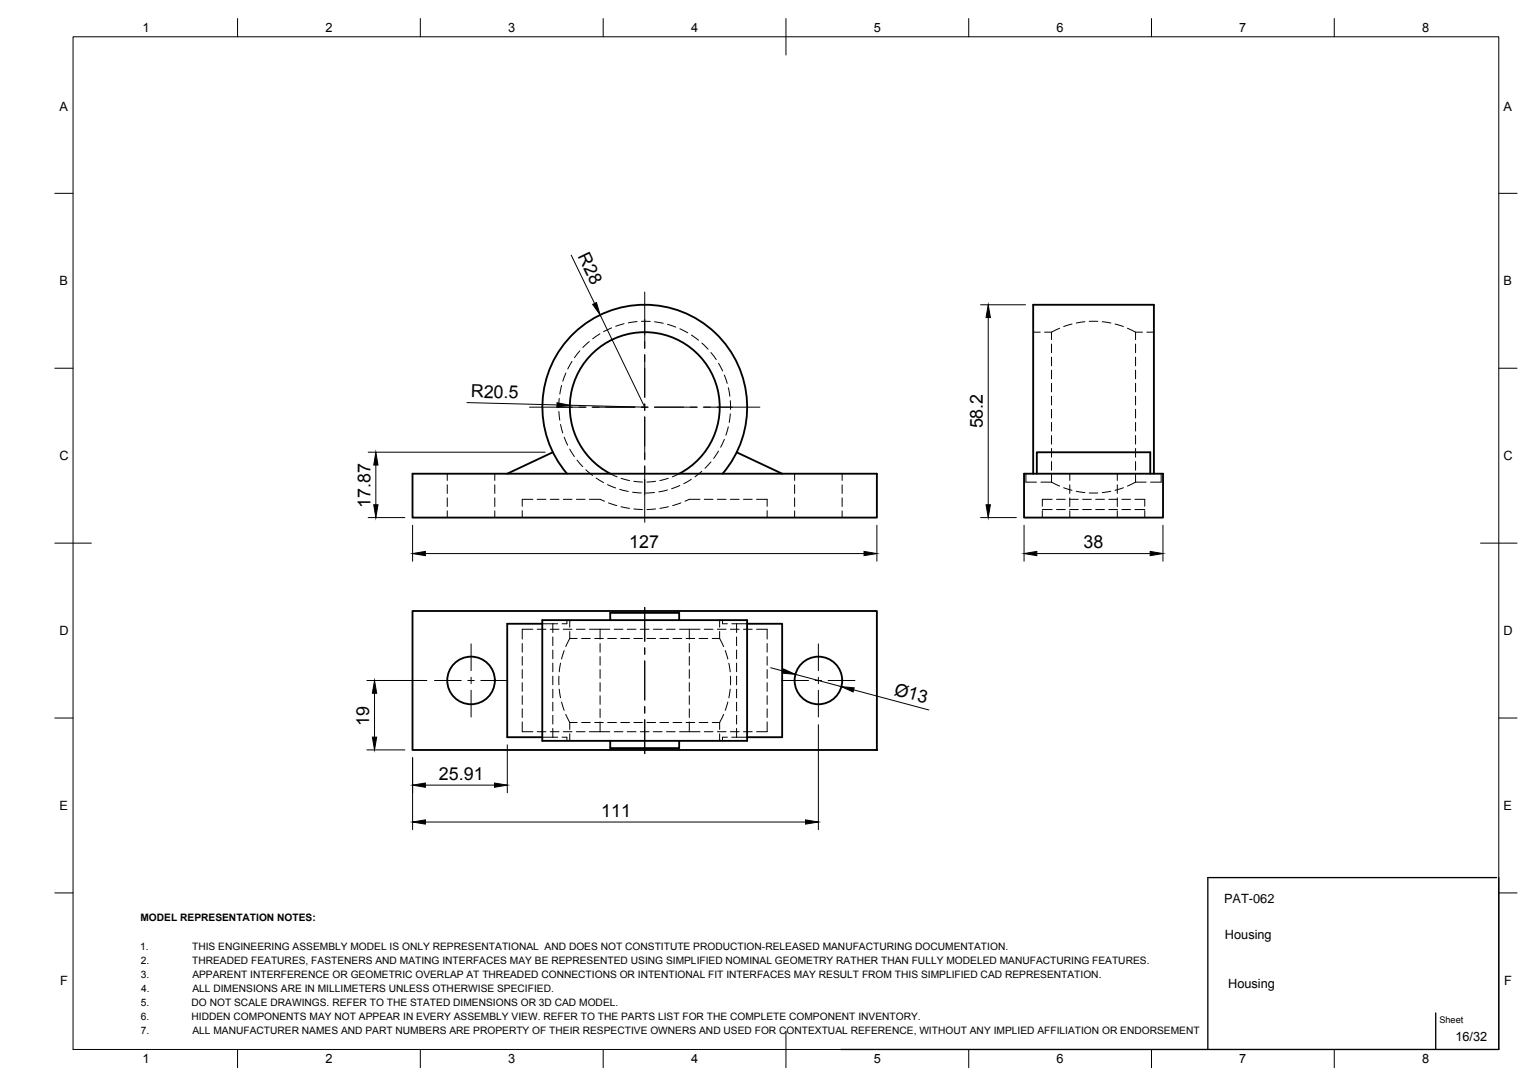
ISO-10303-21;
HEADER;
/* Generated by software containing ST-Developer
 * from STEP Tools, Inc. (www.steptools.com) 
 */

FILE_DESCRIPTION(
/* description */ ('Jaw-coupled motor to shaft test stand'),
/* implementation_level */ '2;1');

FILE_NAME(
/* name */ 'Housing.step',
/* time_stamp */ '2026-10-27T10:46:06-07:00',
/* author */ (''),
/* organization */ (''),
/* preprocessor_version */ 'ST-DEVELOPER v20.2',
/* originating_system */ 'Autodesk Translation Framework v15.17.0.0',
/* authorisation */ '');

FILE_SCHEMA (('AUTOMOTIVE_DESIGN { 1 0 10303 214 3 1 1 }'));
ENDSEC;

DATA;
#10=MECHANICAL_DESIGN_GEOMETRIC_PRESENTATION_REPRESENTATION('',(#353),#19361);
#274=SPHERICAL_SURFACE('',#11594,2.35);
#289=SHAPE_REPRESENTATION_RELATIONSHIP('SRR','None',#19504,#321);
#321=ADVANCED_BREP_SHAPE_REPRESENTATION('',(#386),#19340);
#353=STYLED_ITEM('',(#19725),#386);
#386=MANIFOLD_SOLID_BREP('Body1',#10997);
#452=FACE_BOUND('',#1817,.T.);
#453=FACE_BOUND('',#1818,.T.);
#454=FACE_BOUND('',#1826,.T.);
#455=FACE_BOUND('',#1827,.T.);
#456=FACE_BOUND('',#1828,.T.);
#457=FACE_BOUND('',#1845,.T.);
#458=FACE_BOUND('',#1846,.T.);
#459=FACE_BOUND('',#1847,.T.);
#601=PLANE('',#11580);
#602=PLANE('',#11591);
#603=PLANE('',#11592);
#604=PLANE('',#11596);
#605=PLANE('',#11598);
#606=PLANE('',#11600);
#607=PLANE('',#11602);
#608=PLANE('',#11603);
#609=PLANE('',#11605);
#610=PLANE('',#11606);
#611=PLANE('',#11614);
#612=PLANE('',#11615);
#613=PLANE('',#11616);
#614=PLANE('',#11617);
#615=PLANE('',#11618);
#616=PLANE('',#11619);
#617=PLANE('',#11620);
#618=PLANE('',#11625);
#619=PLANE('',#11626);
#620=PLANE('',#11627);
#621=PLANE('',#11628);
#622=PLANE('',#11629);
#1142=FACE_OUTER_BOUND('',#1811,.T.);
#1143=FACE_OUTER_BOUND('',#1812,.T.);
#1144=FACE_OUTER_BOUND('',#1813,.T.);
#1145=FACE_OUTER_BOUND('',#1814,.T.);
#1146=FACE_OUTER_BOUND('',#1815,.T.);
#1147=FACE_OUTER_BOUND('',#1816,.T.);
#1148=FACE_OUTER_BOUND('',#1819,.T.);
#1149=FACE_OUTER_BOUND('',#1820,.T.);
#1150=FACE_OUTER_BOUND('',#1821,.T.);
#1151=FACE_OUTER_BOUND('',#1822,.T.);
#1152=FACE_OUTER_BOUND('',#1823,.T.);
#1153=FACE_OUTER_BOUND('',#1824,.T.);
#1154=FACE_OUTER_BOUND('',#1825,.T.);
#1155=FACE_OUTER_BOUND('',#1829,.T.);
#1156=FACE_OUTER_BOUND('',#1830,.T.);
#1157=FACE_OUTER_BOUND('',#1831,.T.);
#1158=FACE_OUTER_BOUND('',#1832,.T.);
#1159=FACE_OUTER_BOUND('',#1833,.T.);
#1160=FACE_OUTER_BOUND('',#1834,.T.);
#1161=FACE_OUTER_BOUND('',#1835,.T.);
#1162=FACE_OUTER_BOUND('',#1836,.T.);
#1163=FACE_OUTER_BOUND('',#1837,.T.);
#1164=FACE_OUTER_BOUND('',#1838,.T.);
#1165=FACE_OUTER_BOUND('',#1839,.T.);
#1166=FACE_OUTER_BOUND('',#1840,.T.);
#1167=FACE_OUTER_BOUND('',#1841,.T.);
#1168=FACE_OUTER_BOUND('',#1842,.T.);
#1169=FACE_OUTER_BOUND('',#1843,.T.);
#1170=FACE_OUTER_BOUND('',#1844,.T.);
#1811=EDGE_LOOP('',(#7832,#7833));
#1812=EDGE_LOOP('',(#7834,#7835,#7836,#7837,#7838,#7839,#7840,#7841));
#1813=EDGE_LOOP('',(#7842,#7843,#7844,#7845,#7846,#7847,#7848,#7849));
#1814=EDGE_LOOP('',(#7850,#7851));
#1815=EDGE_LOOP('',(#7852,#7853,#7854,#7855,#7856));
#1816=EDGE_LOOP('',(#7857,#7858));
#1817=EDGE_LOOP('',(#7859));
#1818=EDGE_LOOP('',(#7860));
#1819=EDGE_LOOP('',(#7861,#7862,#7863));
#1820=EDGE_LOOP('',(#7864,#7865,#7866));
#1821=EDGE_LOOP('',(#7867,#7868,#7869));
#1822=EDGE_LOOP('',(#7870,#7871,#7872,#7873));
#1823=EDGE_LOOP('',(#7874,#7875,#7876));
#1824=EDGE_LOOP('',(#7877,#7878,#7879,#7880));
#1825=EDGE_LOOP('',(#7881,#7882,#7883,#7884));
#1826=EDGE_LOOP('',(#7885,#7886,#7887,#7888,#7889,#7890,#7891,#7892,#7893,
#7894,#7895,#7896,#7897,#7898,#7899,#7900,#7901,#7902,#7903,#7904));
#1827=EDGE_LOOP('',(#7905));
#1828=EDGE_LOOP('',(#7906));
#1829=EDGE_LOOP('',(#7907,#7908,#7909,#7910));
#1830=EDGE_LOOP('',(#7911,#7912,#7913,#7914,#7915,#7916,#7917,#7918,#7919,
#7920,#7921,#7922));
#1831=EDGE_LOOP('',(#7923,#7924,#7925,#7926,#7927));
#1832=EDGE_LOOP('',(#7928,#7929,#7930,#7931,#7932,#7933));
#1833=EDGE_LOOP('',(#7934,#7935,#7936,#7937));
#1834=EDGE_LOOP('',(#7938,#7939,#7940,#7941));
#1835=EDGE_LOOP('',(#7942,#7943,#7944,#7945,#7946,#7947));
#1836=EDGE_LOOP('',(#7948,#7949,#7950,#7951));
#1837=EDGE_LOOP('',(#7952,#7953,#7954,#7955));
#1838=EDGE_LOOP('',(#7956,#7957,#7958,#7959));
#1839=EDGE_LOOP('',(#7960,#7961,#7962,#7963));
#1840=EDGE_LOOP('',(#7964,#7965,#7966,#7967));
#1841=EDGE_LOOP('',(#7968,#7969,#7970,#7971));
#1842=EDGE_LOOP('',(#7972,#7973,#7974,#7975));
#1843=EDGE_LOOP('',(#7976,#7977,#7978,#7979));
#1844=EDGE_LOOP('',(#7980,#7981,#7982,#7983));
#1845=EDGE_LOOP('',(#7984,#7985,#7986,#7987));
#1846=EDGE_LOOP('',(#7988));
#1847=EDGE_LOOP('',(#7989));
#2548=LINE('',#15972,#3701);
#2549=LINE('',#15977,#3702);
#2550=LINE('',#15981,#3703);
#2551=LINE('',#15985,#3704);
#2552=LINE('',#15992,#3705);
#2553=LINE('',#15995,#3706);
#2554=LINE('',#15997,#3707);
#2555=LINE('',#16000,#3708);
#2556=LINE('',#16003,#3709);
#2557=LINE('',#16006,#3710);
#2558=LINE('',#16014,#3711);
#2559=LINE('',#16016,#3712);
#2560=LINE('',#16021,#3713);
#2561=LINE('',#16024,#3714);
#2562=LINE('',#16028,#3715);
#2563=LINE('',#16031,#3716);
#2564=LINE('',#16033,#3717);
#2565=LINE('',#16034,#3718);
#2566=LINE('',#16038,#3719);
#2567=LINE('',#16040,#3720);
#2568=LINE('',#16043,#3721);
#2569=LINE('',#16044,#3722);
#2570=LINE('',#16048,#3723);
#2571=LINE('',#16050,#3724);
#2572=LINE('',#16052,#3725);
#2573=LINE('',#16053,#3726);
#2574=LINE('',#16054,#3727);
#2575=LINE('',#16056,#3728);
#2576=LINE('',#16057,#3729);
#2577=LINE('',#16059,#3730);
#2578=LINE('',#16060,#3731);
#2579=LINE('',#16061,#3732);
#2580=LINE('',#16071,#3733);
#2581=LINE('',#16074,#3734);
#2582=LINE('',#16080,#3735);
#2583=LINE('',#16082,#3736);
#2584=LINE('',#16084,#3737);
#2585=LINE('',#16086,#3738);
#2586=LINE('',#16087,#3739);
#2587=LINE('',#16090,#3740);
#2588=LINE('',#16091,#3741);
#2589=LINE('',#16094,#3742);
#2590=LINE('',#16096,#3743);
#2591=LINE('',#16097,#3744);
#2592=LINE('',#16099,#3745);
#2593=LINE('',#16101,#3746);
#2594=LINE('',#16102,#3747);
#2595=LINE('',#16104,#3748);
#2596=LINE('',#16109,#3749);
#2597=LINE('',#16113,#3750);
#2598=LINE('',#16117,#3751);
#2599=LINE('',#16118,#3752);
#2600=LINE('',#16119,#3753);
#2601=LINE('',#16122,#3754);
#2602=LINE('',#16123,#3755);
#2603=LINE('',#16126,#3756);
#2604=LINE('',#16127,#3757);
#2605=LINE('',#16129,#3758);
#3701=VECTOR('',#12929,1.);
#3702=VECTOR('',#12934,1.);
#3703=VECTOR('',#12937,1.);
#3704=VECTOR('',#12940,2.05);
#3705=VECTOR('',#12949,2.05);
#3706=VECTOR('',#12952,1.);
#3707=VECTOR('',#12953,1.);
#3708=VECTOR('',#12958,1.);
#3709=VECTOR('',#12961,1.);
#3710=VECTOR('',#12964,1.);
#3711=VECTOR('',#12971,1.);
#3712=VECTOR('',#12972,1.);
#3713=VECTOR('',#12977,1.);
#3714=VECTOR('',#12980,1.);
#3715=VECTOR('',#12983,1.);
#3716=VECTOR('',#12986,1.);
#3717=VECTOR('',#12989,1.);
#3718=VECTOR('',#12990,1.);
#3719=VECTOR('',#12993,1.);
#3720=VECTOR('',#12994,1.);
#3721=VECTOR('',#12999,1.);
#3722=VECTOR('',#13000,1.);
#3723=VECTOR('',#13003,1.);
#3724=VECTOR('',#13004,1.);
#3725=VECTOR('',#13005,1.);
#3726=VECTOR('',#13006,1.);
#3727=VECTOR('',#13007,1.);
#3728=VECTOR('',#13008,1.);
#3729=VECTOR('',#13009,1.);
#3730=VECTOR('',#13010,1.);
#3731=VECTOR('',#13011,1.);
#3732=VECTOR('',#13012,1.);
#3733=VECTOR('',#13021,1.);
#3734=VECTOR('',#13024,1.);
#3735=VECTOR('',#13033,1.);
#3736=VECTOR('',#13034,1.);
#3737=VECTOR('',#13035,1.);
#3738=VECTOR('',#13036,1.);
#3739=VECTOR('',#13037,1.);
#3740=VECTOR('',#13040,1.);
#3741=VECTOR('',#13041,1.);
#3742=VECTOR('',#13044,1.);
#3743=VECTOR('',#13045,1.);
#3744=VECTOR('',#13046,1.);
#3745=VECTOR('',#13049,1.);
#3746=VECTOR('',#13050,1.);
#3747=VECTOR('',#13051,1.);
#3748=VECTOR('',#13054,1.);
#3749=VECTOR('',#13061,0.65);
#3750=VECTOR('',#13066,0.65);
#3751=VECTOR('',#13069,1.);
#3752=VECTOR('',#13070,1.);
#3753=VECTOR('',#13071,1.);
#3754=VECTOR('',#13074,1.);
#3755=VECTOR('',#13075,1.);
#3756=VECTOR('',#13078,1.);
#3757=VECTOR('',#13079,1.);
#3758=VECTOR('',#13082,1.);
#4751=CIRCLE('',#11581,2.05);
#4752=CIRCLE('',#11583,2.05);
#4753=CIRCLE('',#11584,2.05);
#4754=CIRCLE('',#11585,2.05);
#4755=CIRCLE('',#11586,2.05);
#4756=CIRCLE('',#11588,2.05);
#4757=CIRCLE('',#11589,2.05);
#4758=CIRCLE('',#11590,2.05);
#4759=CIRCLE('',#11593,2.8);
#4760=CIRCLE('',#11595,2.35);
#4761=CIRCLE('',#11597,2.8);
#4762=CIRCLE('',#11599,2.8);
#4763=CIRCLE('',#11601,2.8);
#4764=CIRCLE('',#11604,2.8);
#4765=CIRCLE('',#11607,0.65);
#4766=CIRCLE('',#11608,0.65);
#4767=CIRCLE('',#11610,2.8);
#4768=CIRCLE('',#11611,2.8);
#4769=CIRCLE('',#11613,2.8);
#4770=CIRCLE('',#11622,0.65);
#4771=CIRCLE('',#11624,0.65);
#5105=VERTEX_POINT('',#15970);
#5106=VERTEX_POINT('',#15971);
#5107=VERTEX_POINT('',#15975);
#5108=VERTEX_POINT('',#15976);
#5109=VERTEX_POINT('',#15978);
#5110=VERTEX_POINT('',#15980);
#5111=VERTEX_POINT('',#15982);
#5112=VERTEX_POINT('',#15984);
#5113=VERTEX_POINT('',#15989);
#5114=VERTEX_POINT('',#15991);
#5115=VERTEX_POINT('',#15993);
#5116=VERTEX_POINT('',#15996);
#5117=VERTEX_POINT('',#16002);
#5118=VERTEX_POINT('',#16004);
#5119=VERTEX_POINT('',#16008);
#5120=VERTEX_POINT('',#16009);
#5121=VERTEX_POINT('',#16012);
#5122=VERTEX_POINT('',#16013);
#5123=VERTEX_POINT('',#16015);
#5124=VERTEX_POINT('',#16019);
#5125=VERTEX_POINT('',#16020);
#5126=VERTEX_POINT('',#16022);
#5127=VERTEX_POINT('',#16026);
#5128=VERTEX_POINT('',#16027);
#5129=VERTEX_POINT('',#16029);
#5130=VERTEX_POINT('',#16036);
#5131=VERTEX_POINT('',#16037);
#5132=VERTEX_POINT('',#16039);
#5133=VERTEX_POINT('',#16046);
#5134=VERTEX_POINT('',#16047);
#5135=VERTEX_POINT('',#16049);
#5136=VERTEX_POINT('',#16051);
#5137=VERTEX_POINT('',#16055);
#5138=VERTEX_POINT('',#16058);
#5139=VERTEX_POINT('',#16062);
#5140=VERTEX_POINT('',#16064);
#5141=VERTEX_POINT('',#16067);
#5142=VERTEX_POINT('',#16068);
#5143=VERTEX_POINT('',#16070);
#5144=VERTEX_POINT('',#16072);
#5145=VERTEX_POINT('',#16079);
#5146=VERTEX_POINT('',#16081);
#5147=VERTEX_POINT('',#16083);
#5148=VERTEX_POINT('',#16085);
#5149=VERTEX_POINT('',#16089);
#5150=VERTEX_POINT('',#16093);
#5151=VERTEX_POINT('',#16095);
#5152=VERTEX_POINT('',#16100);
#5153=VERTEX_POINT('',#16107);
#5154=VERTEX_POINT('',#16111);
#5155=VERTEX_POINT('',#16115);
#5156=VERTEX_POINT('',#16116);
#5157=VERTEX_POINT('',#16121);
#5158=VERTEX_POINT('',#16125);
#6127=EDGE_CURVE('',#5105,#5106,#2548,.T.);
#6128=EDGE_CURVE('',#5106,#5105,#4751,.T.);
#6129=EDGE_CURVE('',#5107,#5108,#2549,.T.);
#6130=EDGE_CURVE('',#5107,#5109,#4752,.T.);
#6131=EDGE_CURVE('',#5110,#5109,#2550,.T.);
#6132=EDGE_CURVE('',#5111,#5110,#4753,.T.);
#6133=EDGE_CURVE('',#5111,#5112,#2551,.T.);
#6134=EDGE_CURVE('',#5112,#5112,#4754,.T.);
#6135=EDGE_CURVE('',#5108,#5111,#4755,.T.);
#6136=EDGE_CURVE('',#5113,#5113,#4756,.T.);
#6137=EDGE_CURVE('',#5113,#5114,#2552,.T.);
#6138=EDGE_CURVE('',#5115,#5114,#4757,.T.);
#6139=EDGE_CURVE('',#5106,#5115,#2553,.T.);
#6140=EDGE_CURVE('',#5116,#5105,#2554,.T.);
#6141=EDGE_CURVE('',#5114,#5116,#4758,.T.);
#6142=EDGE_CURVE('',#5109,#5107,#2555,.T.);
#6143=EDGE_CURVE('',#5117,#5110,#2556,.T.);
#6144=EDGE_CURVE('',#5117,#5118,#4759,.T.);
#6145=EDGE_CURVE('',#5108,#5118,#2557,.T.);
#6146=EDGE_CURVE('',#5119,#5120,#4760,.T.);
#6147=EDGE_CURVE('',#5121,#5122,#2558,.T.);
#6148=EDGE_CURVE('',#5121,#5123,#2559,.T.);
#6149=EDGE_CURVE('',#5122,#5123,#4761,.T.);
#6150=EDGE_CURVE('',#5124,#5125,#2560,.T.);
#6151=EDGE_CURVE('',#5126,#5124,#4762,.T.);
#6152=EDGE_CURVE('',#5126,#5125,#2561,.T.);
#6153=EDGE_CURVE('',#5127,#5128,#2562,.T.);
#6154=EDGE_CURVE('',#5129,#5127,#4763,.T.);
#6155=EDGE_CURVE('',#5129,#5128,#2563,.T.);
#6156=EDGE_CURVE('',#5128,#5121,#2564,.T.);
#6157=EDGE_CURVE('',#5123,#5129,#2565,.T.);
#6158=EDGE_CURVE('',#5130,#5131,#2566,.T.);
#6159=EDGE_CURVE('',#5130,#5132,#2567,.T.);
#6160=EDGE_CURVE('',#5131,#5132,#4764,.T.);
#6161=EDGE_CURVE('',#5125,#5130,#2568,.T.);
#6162=EDGE_CURVE('',#5132,#5126,#2569,.T.);
#6163=EDGE_CURVE('',#5133,#5134,#2570,.T.);
#6164=EDGE_CURVE('',#5134,#5135,#2571,.T.);
#6165=EDGE_CURVE('',#5135,#5136,#2572,.T.);
#6166=EDGE_CURVE('',#5136,#5133,#2573,.T.);
#6167=EDGE_CURVE('',#5118,#5127,#2574,.T.);
#6168=EDGE_CURVE('',#5122,#5137,#2575,.T.);
#6169=EDGE_CURVE('',#5137,#5116,#2576,.T.);
#6170=EDGE_CURVE('',#5115,#5138,#2577,.T.);
#6171=EDGE_CURVE('',#5138,#5124,#2578,.T.);
#6172=EDGE_CURVE('',#5131,#5117,#2579,.T.);
#6173=EDGE_CURVE('',#5139,#5139,#4765,.T.);
#6174=EDGE_CURVE('',#5140,#5140,#4766,.T.);
#6175=EDGE_CURVE('',#5141,#5142,#4767,.T.);
#6176=EDGE_CURVE('',#5143,#5141,#2580,.T.);
#6177=EDGE_CURVE('',#5144,#5143,#4768,.T.);
#6178=EDGE_CURVE('',#5142,#5144,#2581,.T.);
#6179=EDGE_CURVE('',#5137,#5138,#4769,.T.);
#6180=EDGE_CURVE('',#5143,#5145,#2582,.T.);
#6181=EDGE_CURVE('',#5146,#5145,#2583,.T.);
#6182=EDGE_CURVE('',#5147,#5146,#2584,.T.);
#6183=EDGE_CURVE('',#5147,#5148,#2585,.T.);
#6184=EDGE_CURVE('',#5148,#5144,#2586,.T.);
#6185=EDGE_CURVE('',#5149,#5141,#2587,.T.);
#6186=EDGE_CURVE('',#5145,#5149,#2588,.T.);
#6187=EDGE_CURVE('',#5150,#5147,#2589,.T.);
#6188=EDGE_CURVE('',#5150,#5151,#2590,.T.);
#6189=EDGE_CURVE('',#5151,#5148,#2591,.T.);
#6190=EDGE_CURVE('',#5142,#5151,#2592,.T.);
#6191=EDGE_CURVE('',#5152,#5150,#2593,.T.);
#6192=EDGE_CURVE('',#5152,#5149,#2594,.T.);
#6193=EDGE_CURVE('',#5146,#5152,#2595,.T.);
#6194=EDGE_CURVE('',#5153,#5153,#4770,.T.);
#6195=EDGE_CURVE('',#5153,#5140,#2596,.T.);
#6196=EDGE_CURVE('',#5154,#5154,#4771,.T.);
#6197=EDGE_CURVE('',#5154,#5139,#2597,.T.);
#6198=EDGE_CURVE('',#5155,#5156,#2598,.T.);
#6199=EDGE_CURVE('',#5156,#5133,#2599,.T.);
#6200=EDGE_CURVE('',#5155,#5136,#2600,.T.);
#6201=EDGE_CURVE('',#5157,#5155,#2601,.T.);
#6202=EDGE_CURVE('',#5157,#5135,#2602,.T.);
#6203=EDGE_CURVE('',#5158,#5157,#2603,.T.);
#6204=EDGE_CURVE('',#5158,#5134,#2604,.T.);
#6205=EDGE_CURVE('',#5156,#5158,#2605,.T.);
#7832=ORIENTED_EDGE('',*,*,#6127,.F.);
#7833=ORIENTED_EDGE('',*,*,#6128,.F.);
#7834=ORIENTED_EDGE('',*,*,#6129,.F.);
#7835=ORIENTED_EDGE('',*,*,#6130,.T.);
#7836=ORIENTED_EDGE('',*,*,#6131,.F.);
#7837=ORIENTED_EDGE('',*,*,#6132,.F.);
#7838=ORIENTED_EDGE('',*,*,#6133,.T.);
#7839=ORIENTED_EDGE('',*,*,#6134,.F.);
#7840=ORIENTED_EDGE('',*,*,#6133,.F.);
#7841=ORIENTED_EDGE('',*,*,#6135,.F.);
#7842=ORIENTED_EDGE('',*,*,#6136,.F.);
#7843=ORIENTED_EDGE('',*,*,#6137,.T.);
#7844=ORIENTED_EDGE('',*,*,#6138,.F.);
#7845=ORIENTED_EDGE('',*,*,#6139,.F.);
#7846=ORIENTED_EDGE('',*,*,#6128,.T.);
#7847=ORIENTED_EDGE('',*,*,#6140,.F.);
#7848=ORIENTED_EDGE('',*,*,#6141,.F.);
#7849=ORIENTED_EDGE('',*,*,#6137,.F.);
#7850=ORIENTED_EDGE('',*,*,#6142,.F.);
#7851=ORIENTED_EDGE('',*,*,#6130,.F.);
#7852=ORIENTED_EDGE('',*,*,#6135,.T.);
#7853=ORIENTED_EDGE('',*,*,#6132,.T.);
#7854=ORIENTED_EDGE('',*,*,#6143,.F.);
#7855=ORIENTED_EDGE('',*,*,#6144,.T.);
#7856=ORIENTED_EDGE('',*,*,#6145,.F.);
#7857=ORIENTED_EDGE('',*,*,#6146,.T.);
#7858=ORIENTED_EDGE('',*,*,#6146,.F.);
#7859=ORIENTED_EDGE('',*,*,#6136,.T.);
#7860=ORIENTED_EDGE('',*,*,#6134,.T.);
#7861=ORIENTED_EDGE('',*,*,#6147,.F.);
#7862=ORIENTED_EDGE('',*,*,#6148,.T.);
#7863=ORIENTED_EDGE('',*,*,#6149,.F.);
#7864=ORIENTED_EDGE('',*,*,#6150,.F.);
#7865=ORIENTED_EDGE('',*,*,#6151,.F.);
#7866=ORIENTED_EDGE('',*,*,#6152,.T.);
#7867=ORIENTED_EDGE('',*,*,#6153,.F.);
#7868=ORIENTED_EDGE('',*,*,#6154,.F.);
#7869=ORIENTED_EDGE('',*,*,#6155,.T.);
#7870=ORIENTED_EDGE('',*,*,#6156,.F.);
#7871=ORIENTED_EDGE('',*,*,#6155,.F.);
#7872=ORIENTED_EDGE('',*,*,#6157,.F.);
#7873=ORIENTED_EDGE('',*,*,#6148,.F.);
#7874=ORIENTED_EDGE('',*,*,#6158,.F.);
#7875=ORIENTED_EDGE('',*,*,#6159,.T.);
#7876=ORIENTED_EDGE('',*,*,#6160,.F.);
#7877=ORIENTED_EDGE('',*,*,#6161,.F.);
#7878=ORIENTED_EDGE('',*,*,#6152,.F.);
#7879=ORIENTED_EDGE('',*,*,#6162,.F.);
#7880=ORIENTED_EDGE('',*,*,#6159,.F.);
#7881=ORIENTED_EDGE('',*,*,#6163,.T.);
#7882=ORIENTED_EDGE('',*,*,#6164,.T.);
#7883=ORIENTED_EDGE('',*,*,#6165,.T.);
#7884=ORIENTED_EDGE('',*,*,#6166,.T.);
#7885=ORIENTED_EDGE('',*,*,#6129,.T.);
#7886=ORIENTED_EDGE('',*,*,#6145,.T.);
#7887=ORIENTED_EDGE('',*,*,#6167,.T.);
#7888=ORIENTED_EDGE('',*,*,#6153,.T.);
#7889=ORIENTED_EDGE('',*,*,#6156,.T.);
#7890=ORIENTED_EDGE('',*,*,#6147,.T.);
#7891=ORIENTED_EDGE('',*,*,#6168,.T.);
#7892=ORIENTED_EDGE('',*,*,#6169,.T.);
#7893=ORIENTED_EDGE('',*,*,#6140,.T.);
#7894=ORIENTED_EDGE('',*,*,#6127,.T.);
#7895=ORIENTED_EDGE('',*,*,#6139,.T.);
#7896=ORIENTED_EDGE('',*,*,#6170,.T.);
#7897=ORIENTED_EDGE('',*,*,#6171,.T.);
#7898=ORIENTED_EDGE('',*,*,#6150,.T.);
#7899=ORIENTED_EDGE('',*,*,#6161,.T.);
#7900=ORIENTED_EDGE('',*,*,#6158,.T.);
#7901=ORIENTED_EDGE('',*,*,#6172,.T.);
#7902=ORIENTED_EDGE('',*,*,#6143,.T.);
#7903=ORIENTED_EDGE('',*,*,#6131,.T.);
#7904=ORIENTED_EDGE('',*,*,#6142,.T.);
#7905=ORIENTED_EDGE('',*,*,#6173,.T.);
#7906=ORIENTED_EDGE('',*,*,#6174,.T.);
#7907=ORIENTED_EDGE('',*,*,#6175,.F.);
#7908=ORIENTED_EDGE('',*,*,#6176,.F.);
#7909=ORIENTED_EDGE('',*,*,#6177,.F.);
#7910=ORIENTED_EDGE('',*,*,#6178,.F.);
#7911=ORIENTED_EDGE('',*,*,#6151,.T.);
#7912=ORIENTED_EDGE('',*,*,#6171,.F.);
#7913=ORIENTED_EDGE('',*,*,#6179,.F.);
#7914=ORIENTED_EDGE('',*,*,#6168,.F.);
#7915=ORIENTED_EDGE('',*,*,#6149,.T.);
#7916=ORIENTED_EDGE('',*,*,#6157,.T.);
#7917=ORIENTED_EDGE('',*,*,#6154,.T.);
#7918=ORIENTED_EDGE('',*,*,#6167,.F.);
#7919=ORIENTED_EDGE('',*,*,#6144,.F.);
#7920=ORIENTED_EDGE('',*,*,#6172,.F.);
#7921=ORIENTED_EDGE('',*,*,#6160,.T.);
#7922=ORIENTED_EDGE('',*,*,#6162,.T.);
#7923=ORIENTED_EDGE('',*,*,#6138,.T.);
#7924=ORIENTED_EDGE('',*,*,#6141,.T.);
#7925=ORIENTED_EDGE('',*,*,#6169,.F.);
#7926=ORIENTED_EDGE('',*,*,#6179,.T.);
#7927=ORIENTED_EDGE('',*,*,#6170,.F.);
#7928=ORIENTED_EDGE('',*,*,#6177,.T.);
#7929=ORIENTED_EDGE('',*,*,#6180,.T.);
#7930=ORIENTED_EDGE('',*,*,#6181,.F.);
#7931=ORIENTED_EDGE('',*,*,#6182,.F.);
#7932=ORIENTED_EDGE('',*,*,#6183,.T.);
#7933=ORIENTED_EDGE('',*,*,#6184,.T.);
#7934=ORIENTED_EDGE('',*,*,#6176,.T.);
#7935=ORIENTED_EDGE('',*,*,#6185,.F.);
#7936=ORIENTED_EDGE('',*,*,#6186,.F.);
#7937=ORIENTED_EDGE('',*,*,#6180,.F.);
#7938=ORIENTED_EDGE('',*,*,#6187,.F.);
#7939=ORIENTED_EDGE('',*,*,#6188,.T.);
#7940=ORIENTED_EDGE('',*,*,#6189,.T.);
#7941=ORIENTED_EDGE('',*,*,#6183,.F.);
#7942=ORIENTED_EDGE('',*,*,#6175,.T.);
#7943=ORIENTED_EDGE('',*,*,#6190,.T.);
#7944=ORIENTED_EDGE('',*,*,#6188,.F.);
#7945=ORIENTED_EDGE('',*,*,#6191,.F.);
#7946=ORIENTED_EDGE('',*,*,#6192,.T.);
#7947=ORIENTED_EDGE('',*,*,#6185,.T.);
#7948=ORIENTED_EDGE('',*,*,#6193,.F.);
#7949=ORIENTED_EDGE('',*,*,#6181,.T.);
#7950=ORIENTED_EDGE('',*,*,#6186,.T.);
#7951=ORIENTED_EDGE('',*,*,#6192,.F.);
#7952=ORIENTED_EDGE('',*,*,#6178,.T.);
#7953=ORIENTED_EDGE('',*,*,#6184,.F.);
#7954=ORIENTED_EDGE('',*,*,#6189,.F.);
#7955=ORIENTED_EDGE('',*,*,#6190,.F.);
#7956=ORIENTED_EDGE('',*,*,#6194,.F.);
#7957=ORIENTED_EDGE('',*,*,#6195,.T.);
#7958=ORIENTED_EDGE('',*,*,#6174,.F.);
#7959=ORIENTED_EDGE('',*,*,#6195,.F.);
#7960=ORIENTED_EDGE('',*,*,#6196,.F.);
#7961=ORIENTED_EDGE('',*,*,#6197,.T.);
#7962=ORIENTED_EDGE('',*,*,#6173,.F.);
#7963=ORIENTED_EDGE('',*,*,#6197,.F.);
#7964=ORIENTED_EDGE('',*,*,#6198,.T.);
#7965=ORIENTED_EDGE('',*,*,#6199,.T.);
#7966=ORIENTED_EDGE('',*,*,#6166,.F.);
#7967=ORIENTED_EDGE('',*,*,#6200,.F.);
#7968=ORIENTED_EDGE('',*,*,#6201,.T.);
#7969=ORIENTED_EDGE('',*,*,#6200,.T.);
#7970=ORIENTED_EDGE('',*,*,#6165,.F.);
#7971=ORIENTED_EDGE('',*,*,#6202,.F.);
#7972=ORIENTED_EDGE('',*,*,#6203,.T.);
#7973=ORIENTED_EDGE('',*,*,#6202,.T.);
#7974=ORIENTED_EDGE('',*,*,#6164,.F.);
#7975=ORIENTED_EDGE('',*,*,#6204,.F.);
#7976=ORIENTED_EDGE('',*,*,#6205,.T.);
#7977=ORIENTED_EDGE('',*,*,#6204,.T.);
#7978=ORIENTED_EDGE('',*,*,#6163,.F.);
#7979=ORIENTED_EDGE('',*,*,#6199,.F.);
#7980=ORIENTED_EDGE('',*,*,#6205,.F.);
#7981=ORIENTED_EDGE('',*,*,#6198,.F.);
#7982=ORIENTED_EDGE('',*,*,#6201,.F.);
#7983=ORIENTED_EDGE('',*,*,#6203,.F.);
#7984=ORIENTED_EDGE('',*,*,#6182,.T.);
#7985=ORIENTED_EDGE('',*,*,#6193,.T.);
#7986=ORIENTED_EDGE('',*,*,#6191,.T.);
#7987=ORIENTED_EDGE('',*,*,#6187,.T.);
#7988=ORIENTED_EDGE('',*,*,#6194,.T.);
#7989=ORIENTED_EDGE('',*,*,#6196,.T.);
#10305=CYLINDRICAL_SURFACE('',#11582,2.05);
#10306=CYLINDRICAL_SURFACE('',#11587,2.05);
#10307=CYLINDRICAL_SURFACE('',#11609,2.8);
#10308=CYLINDRICAL_SURFACE('',#11612,2.8);
#10309=CYLINDRICAL_SURFACE('',#11621,0.65);
#10310=CYLINDRICAL_SURFACE('',#11623,0.65);
#10484=ADVANCED_FACE('',(#1142),#601,.F.);
#10485=ADVANCED_FACE('',(#1143),#10305,.F.);
#10486=ADVANCED_FACE('',(#1144),#10306,.F.);
#10487=ADVANCED_FACE('',(#1145),#602,.T.);
#10488=ADVANCED_FACE('',(#1146),#603,.F.);
#10489=ADVANCED_FACE('',(#1147,#452,#453),#274,.F.);
#10490=ADVANCED_FACE('',(#1148),#604,.T.);
#10491=ADVANCED_FACE('',(#1149),#605,.T.);
#10492=ADVANCED_FACE('',(#1150),#606,.T.);
#10493=ADVANCED_FACE('',(#1151),#607,.T.);
#10494=ADVANCED_FACE('',(#1152),#608,.T.);
#10495=ADVANCED_FACE('',(#1153),#609,.T.);
#10496=ADVANCED_FACE('',(#1154,#454,#455,#456),#610,.T.);
#10497=ADVANCED_FACE('',(#1155),#10307,.T.);
#10498=ADVANCED_FACE('',(#1156),#10308,.T.);
#10499=ADVANCED_FACE('',(#1157),#611,.T.);
#10500=ADVANCED_FACE('',(#1158),#612,.F.);
#10501=ADVANCED_FACE('',(#1159),#613,.F.);
#10502=ADVANCED_FACE('',(#1160),#614,.F.);
#10503=ADVANCED_FACE('',(#1161),#615,.F.);
#10504=ADVANCED_FACE('',(#1162),#616,.F.);
#10505=ADVANCED_FACE('',(#1163),#617,.F.);
#10506=ADVANCED_FACE('',(#1164),#10309,.F.);
#10507=ADVANCED_FACE('',(#1165),#10310,.F.);
#10508=ADVANCED_FACE('',(#1166),#618,.T.);
#10509=ADVANCED_FACE('',(#1167),#619,.T.);
#10510=ADVANCED_FACE('',(#1168),#620,.T.);
#10511=ADVANCED_FACE('',(#1169),#621,.T.);
#10512=ADVANCED_FACE('',(#1170,#457,#458,#459),#622,.F.);
#10997=CLOSED_SHELL('',(#10484,#10485,#10486,#10487,#10488,#10489,#10490,
#10491,#10492,#10493,#10494,#10495,#10496,#10497,#10498,#10499,#10500,#10501,
#10502,#10503,#10504,#10505,#10506,#10507,#10508,#10509,#10510,#10511,#10512));
#11579=AXIS2_PLACEMENT_3D('',#15968,#12925,#12926);
#11580=AXIS2_PLACEMENT_3D('',#15969,#12927,#12928);
#11581=AXIS2_PLACEMENT_3D('',#15973,#12930,#12931);
#11582=AXIS2_PLACEMENT_3D('',#15974,#12932,#12933);
#11583=AXIS2_PLACEMENT_3D('',#15979,#12935,#12936);
#11584=AXIS2_PLACEMENT_3D('',#15983,#12938,#12939);
#11585=AXIS2_PLACEMENT_3D('',#15986,#12941,#12942);
#11586=AXIS2_PLACEMENT_3D('',#15987,#12943,#12944);
#11587=AXIS2_PLACEMENT_3D('',#15988,#12945,#12946);
#11588=AXIS2_PLACEMENT_3D('',#15990,#12947,#12948);
#11589=AXIS2_PLACEMENT_3D('',#15994,#12950,#12951);
#11590=AXIS2_PLACEMENT_3D('',#15998,#12954,#12955);
#11591=AXIS2_PLACEMENT_3D('',#15999,#12956,#12957);
#11592=AXIS2_PLACEMENT_3D('',#16001,#12959,#12960);
#11593=AXIS2_PLACEMENT_3D('',#16005,#12962,#12963);
#11594=AXIS2_PLACEMENT_3D('',#16007,#12965,#12966);
#11595=AXIS2_PLACEMENT_3D('',#16010,#12967,#12968);
#11596=AXIS2_PLACEMENT_3D('',#16011,#12969,#12970);
#11597=AXIS2_PLACEMENT_3D('',#16017,#12973,#12974);
#11598=AXIS2_PLACEMENT_3D('',#16018,#12975,#12976);
#11599=AXIS2_PLACEMENT_3D('',#16023,#12978,#12979);
#11600=AXIS2_PLACEMENT_3D('',#16025,#12981,#12982);
#11601=AXIS2_PLACEMENT_3D('',#16030,#12984,#12985);
#11602=AXIS2_PLACEMENT_3D('',#16032,#12987,#12988);
#11603=AXIS2_PLACEMENT_3D('',#16035,#12991,#12992);
#11604=AXIS2_PLACEMENT_3D('',#16041,#12995,#12996);
#11605=AXIS2_PLACEMENT_3D('',#16042,#12997,#12998);
#11606=AXIS2_PLACEMENT_3D('',#16045,#13001,#13002);
#11607=AXIS2_PLACEMENT_3D('',#16063,#13013,#13014);
#11608=AXIS2_PLACEMENT_3D('',#16065,#13015,#13016);
#11609=AXIS2_PLACEMENT_3D('',#16066,#13017,#13018);
#11610=AXIS2_PLACEMENT_3D('',#16069,#13019,#13020);
#11611=AXIS2_PLACEMENT_3D('',#16073,#13022,#13023);
#11612=AXIS2_PLACEMENT_3D('',#16075,#13025,#13026);
#11613=AXIS2_PLACEMENT_3D('',#16076,#13027,#13028);
#11614=AXIS2_PLACEMENT_3D('',#16077,#13029,#13030);
#11615=AXIS2_PLACEMENT_3D('',#16078,#13031,#13032);
#11616=AXIS2_PLACEMENT_3D('',#16088,#13038,#13039);
#11617=AXIS2_PLACEMENT_3D('',#16092,#13042,#13043);
#11618=AXIS2_PLACEMENT_3D('',#16098,#13047,#13048);
#11619=AXIS2_PLACEMENT_3D('',#16103,#13052,#13053);
#11620=AXIS2_PLACEMENT_3D('',#16105,#13055,#13056);
#11621=AXIS2_PLACEMENT_3D('',#16106,#13057,#13058);
#11622=AXIS2_PLACEMENT_3D('',#16108,#13059,#13060);
#11623=AXIS2_PLACEMENT_3D('',#16110,#13062,#13063);
#11624=AXIS2_PLACEMENT_3D('',#16112,#13064,#13065);
#11625=AXIS2_PLACEMENT_3D('',#16114,#13067,#13068);
#11626=AXIS2_PLACEMENT_3D('',#16120,#13072,#13073);
#11627=AXIS2_PLACEMENT_3D('',#16124,#13076,#13077);
#11628=AXIS2_PLACEMENT_3D('',#16128,#13080,#13081);
#11629=AXIS2_PLACEMENT_3D('',#16130,#13083,#13084);
#12925=DIRECTION('axis',(0.,0.,1.));
#12926=DIRECTION('refdir',(1.,0.,0.));
#12927=DIRECTION('center_axis',(0.,1.,0.));
#12928=DIRECTION('ref_axis',(1.,0.,0.));
#12929=DIRECTION('',(1.,0.,0.));
#12930=DIRECTION('center_axis',(0.,1.,0.));
#12931=DIRECTION('ref_axis',(1.,0.,0.));
#12932=DIRECTION('center_axis',(0.,1.,0.));
#12933=DIRECTION('ref_axis',(1.,0.,0.));
#12934=DIRECTION('',(0.,1.,0.));
#12935=DIRECTION('center_axis',(0.,-1.,0.));
#12936=DIRECTION('ref_axis',(1.,0.,0.));
#12937=DIRECTION('',(0.,-1.,0.));
#12938=DIRECTION('center_axis',(0.,1.,0.));
#12939=DIRECTION('ref_axis',(1.,0.,0.));
#12940=DIRECTION('',(0.,1.,0.));
#12941=DIRECTION('center_axis',(0.,-1.,0.));
#12942=DIRECTION('ref_axis',(1.,0.,0.));
#12943=DIRECTION('center_axis',(0.,1.,0.));
#12944=DIRECTION('ref_axis',(1.,0.,0.));
#12945=DIRECTION('center_axis',(0.,1.,0.));
#12946=DIRECTION('ref_axis',(1.,0.,0.));
#12947=DIRECTION('center_axis',(0.,1.,0.));
#12948=DIRECTION('ref_axis',(1.,0.,0.));
#12949=DIRECTION('',(0.,1.,0.));
#12950=DIRECTION('center_axis',(0.,-1.,0.));
#12951=DIRECTION('ref_axis',(1.,0.,0.));
#12952=DIRECTION('',(0.,-1.,0.));
#12953=DIRECTION('',(0.,1.,0.));
#12954=DIRECTION('center_axis',(0.,-1.,0.));
#12955=DIRECTION('ref_axis',(1.,0.,0.));
#12956=DIRECTION('center_axis',(0.,1.,0.));
#12957=DIRECTION('ref_axis',(1.,0.,0.));
#12958=DIRECTION('',(-1.,0.,0.));
#12959=DIRECTION('center_axis',(0.,1.,0.));
#12960=DIRECTION('ref_axis',(1.,0.,0.));
#12961=DIRECTION('',(-1.,0.,0.));
#12962=DIRECTION('center_axis',(0.,-1.,0.));
#12963=DIRECTION('ref_axis',(1.,0.,0.));
#12964=DIRECTION('',(-1.,0.,0.));
#12965=DIRECTION('center_axis',(6.12323399573677E-17,0.,1.));
#12966=DIRECTION('ref_axis',(1.,0.,0.));
#12967=DIRECTION('center_axis',(-1.22464679914735E-16,1.,0.));
#12968=DIRECTION('ref_axis',(-1.,-1.22464679914735E-16,0.));
#12969=DIRECTION('center_axis',(0.,1.,0.));
#12970=DIRECTION('ref_axis',(0.,0.,1.));
#12971=DIRECTION('',(1.,0.,0.));
#12972=DIRECTION('',(0.9045256429963,0.,0.426419231698256));
#12973=DIRECTION('center_axis',(0.,1.,0.));
#12974=DIRECTION('ref_axis',(1.,0.,0.));
#12975=DIRECTION('center_axis',(0.,1.,0.));
#12976=DIRECTION('ref_axis',(0.,0.,1.));
#12977=DIRECTION('',(1.,0.,0.));
#12978=DIRECTION('center_axis',(0.,1.,0.));
#12979=DIRECTION('ref_axis',(1.,0.,0.));
#12980=DIRECTION('',(0.9045256429963,0.,-0.426419231698256));
#12981=DIRECTION('center_axis',(0.,-1.,0.));
#12982=DIRECTION('ref_axis',(0.,0.,-1.));
#12983=DIRECTION('',(-1.,0.,0.));
#12984=DIRECTION('center_axis',(0.,-1.,0.));
#12985=DIRECTION('ref_axis',(1.,0.,0.));
#12986=DIRECTION('',(-0.9045256429963,0.,-0.426419231698256));
#12987=DIRECTION('center_axis',(-0.426419231698256,0.,0.9045256429963));
#12988=DIRECTION('ref_axis',(0.9045256429963,0.,0.426419231698256));
#12989=DIRECTION('',(0.,1.,0.));
#12990=DIRECTION('',(0.,-1.,0.));
#12991=DIRECTION('center_axis',(0.,-1.,0.));
#12992=DIRECTION('ref_axis',(0.,0.,-1.));
#12993=DIRECTION('',(-1.,0.,0.));
#12994=DIRECTION('',(-0.9045256429963,0.,0.426419231698256));
#12995=DIRECTION('center_axis',(0.,-1.,0.));
#12996=DIRECTION('ref_axis',(1.,0.,0.));
#12997=DIRECTION('center_axis',(0.426419231698256,0.,0.9045256429963));
#12998=DIRECTION('ref_axis',(0.9045256429963,0.,-0.426419231698256));
#12999=DIRECTION('',(0.,-1.,0.));
#13000=DIRECTION('',(0.,1.,0.));
#13001=DIRECTION('center_axis',(0.,0.,1.));
#13002=DIRECTION('ref_axis',(1.,0.,0.));
#13003=DIRECTION('',(0.,-1.,0.));
#13004=DIRECTION('',(1.,0.,0.));
#13005=DIRECTION('',(0.,1.,0.));
#13006=DIRECTION('',(-1.,0.,0.));
#13007=DIRECTION('',(0.,1.,0.));
#13008=DIRECTION('',(0.,1.,0.));
#13009=DIRECTION('',(1.,0.,0.));
#13010=DIRECTION('',(1.,0.,0.));
#13011=DIRECTION('',(0.,-1.,0.));
#13012=DIRECTION('',(0.,-1.,0.));
#13013=DIRECTION('center_axis',(0.,0.,-1.));
#13014=DIRECTION('ref_axis',(1.,0.,0.));
#13015=DIRECTION('center_axis',(0.,0.,-1.));
#13016=DIRECTION('ref_axis',(1.,0.,0.));
#13017=DIRECTION('center_axis',(0.,1.,0.));
#13018=DIRECTION('ref_axis',(1.,0.,0.));
#13019=DIRECTION('center_axis',(0.,-1.,0.));
#13020=DIRECTION('ref_axis',(1.,0.,0.));
#13021=DIRECTION('',(0.,-1.,0.));
#13022=DIRECTION('center_axis',(0.,1.,0.));
#13023=DIRECTION('ref_axis',(1.,0.,0.));
#13024=DIRECTION('',(0.,1.,0.));
#13025=DIRECTION('center_axis',(0.,1.,0.));
#13026=DIRECTION('ref_axis',(6.12323399573677E-17,0.,1.));
#13027=DIRECTION('center_axis',(0.,1.,0.));
#13028=DIRECTION('ref_axis',(1.,0.,0.));
#13029=DIRECTION('center_axis',(0.,1.,0.));
#13030=DIRECTION('ref_axis',(1.,0.,0.));
#13031=DIRECTION('center_axis',(0.,1.,0.));
#13032=DIRECTION('ref_axis',(-1.,0.,0.));
#13033=DIRECTION('',(-1.,0.,0.));
#13034=DIRECTION('',(0.,0.,1.));
#13035=DIRECTION('',(-1.,0.,0.));
#13036=DIRECTION('',(0.,0.,1.));
#13037=DIRECTION('',(-1.,0.,0.));
#13038=DIRECTION('center_axis',(0.,0.,1.));
#13039=DIRECTION('ref_axis',(1.,0.,0.));
#13040=DIRECTION('',(1.,0.,0.));
#13041=DIRECTION('',(0.,-1.,0.));
#13042=DIRECTION('center_axis',(1.,0.,0.));
#13043=DIRECTION('ref_axis',(0.,1.,0.));
#13044=DIRECTION('',(0.,1.,0.));
#13045=DIRECTION('',(0.,0.,1.));
#13046=DIRECTION('',(0.,1.,0.));
#13047=DIRECTION('center_axis',(0.,-1.,0.));
#13048=DIRECTION('ref_axis',(1.,0.,0.));
#13049=DIRECTION('',(1.,0.,0.));
#13050=DIRECTION('',(1.,0.,0.));
#13051=DIRECTION('',(0.,0.,1.));
#13052=DIRECTION('center_axis',(-1.,0.,0.));
#13053=DIRECTION('ref_axis',(0.,-1.,0.));
#13054=DIRECTION('',(0.,-1.,0.));
#13055=DIRECTION('center_axis',(0.,0.,1.));
#13056=DIRECTION('ref_axis',(1.,0.,0.));
#13057=DIRECTION('center_axis',(0.,0.,1.));
#13058=DIRECTION('ref_axis',(1.,0.,0.));
#13059=DIRECTION('center_axis',(0.,0.,1.));
#13060=DIRECTION('ref_axis',(1.,0.,0.));
#13061=DIRECTION('',(0.,0.,1.));
#13062=DIRECTION('center_axis',(0.,0.,1.));
#13063=DIRECTION('ref_axis',(1.,0.,0.));
#13064=DIRECTION('center_axis',(0.,0.,1.));
#13065=DIRECTION('ref_axis',(1.,0.,0.));
#13066=DIRECTION('',(0.,0.,1.));
#13067=DIRECTION('center_axis',(0.,1.,0.));
#13068=DIRECTION('ref_axis',(-1.,0.,0.));
#13069=DIRECTION('',(-1.,0.,0.));
#13070=DIRECTION('',(0.,0.,1.));
#13071=DIRECTION('',(0.,0.,1.));
#13072=DIRECTION('center_axis',(1.,0.,0.));
#13073=DIRECTION('ref_axis',(0.,1.,0.));
#13074=DIRECTION('',(0.,1.,0.));
#13075=DIRECTION('',(0.,0.,1.));
#13076=DIRECTION('center_axis',(0.,-1.,0.));
#13077=DIRECTION('ref_axis',(1.,0.,0.));
#13078=DIRECTION('',(1.,0.,0.));
#13079=DIRECTION('',(0.,0.,1.));
#13080=DIRECTION('center_axis',(-1.,0.,0.));
#13081=DIRECTION('ref_axis',(0.,-1.,0.));
#13082=DIRECTION('',(0.,-1.,0.));
#13083=DIRECTION('center_axis',(0.,0.,1.));
#13084=DIRECTION('ref_axis',(1.,0.,0.));
#15968=CARTESIAN_POINT('',(0.,0.,0.));
#15969=CARTESIAN_POINT('Origin',(0.,1.85,0.));
#15970=CARTESIAN_POINT('',(-0.943451111610983,1.85,-1.82));
#15971=CARTESIAN_POINT('',(0.943451111610983,1.85,-1.82));
#15972=CARTESIAN_POINT('',(0.,1.85,-1.82));
#15973=CARTESIAN_POINT('Origin',(0.,1.85,0.));
#15974=CARTESIAN_POINT('Origin',(0.,0.,0.));
#15975=CARTESIAN_POINT('',(-0.943451111610983,-1.85,-1.82));
#15976=CARTESIAN_POINT('',(-0.943451111610983,-1.65,-1.82));
#15977=CARTESIAN_POINT('',(-0.943451111610983,0.,-1.82));
#15978=CARTESIAN_POINT('',(0.943451111610983,-1.85,-1.82));
#15979=CARTESIAN_POINT('Origin',(0.,-1.85,0.));
#15980=CARTESIAN_POINT('',(0.943451111610983,-1.65,-1.82));
#15981=CARTESIAN_POINT('',(0.943451111610983,0.,-1.82));
#15982=CARTESIAN_POINT('',(-2.05,-1.65,2.51052593825207E-16));
#15983=CARTESIAN_POINT('Origin',(0.,-1.65,0.));
#15984=CARTESIAN_POINT('',(-2.05,-1.14891252930761,-2.51052593825207E-16));
#15985=CARTESIAN_POINT('',(-2.05,0.,2.51052593825207E-16));
#15986=CARTESIAN_POINT('Origin',(0.,-1.14891252930761,0.));
#15987=CARTESIAN_POINT('Origin',(0.,-1.65,0.));
#15988=CARTESIAN_POINT('Origin',(0.,0.,0.));
#15989=CARTESIAN_POINT('',(-2.05,1.14891252930761,2.51052593825207E-16));
#15990=CARTESIAN_POINT('Origin',(0.,1.14891252930761,0.));
#15991=CARTESIAN_POINT('',(-2.05,1.65,2.51052593825207E-16));
#15992=CARTESIAN_POINT('',(-2.05,0.,2.51052593825207E-16));
#15993=CARTESIAN_POINT('',(0.943451111610983,1.65,-1.82));
#15994=CARTESIAN_POINT('Origin',(0.,1.65,0.));
#15995=CARTESIAN_POINT('',(0.943451111610983,0.,-1.82));
#15996=CARTESIAN_POINT('',(-0.943451111610983,1.65,-1.82));
#15997=CARTESIAN_POINT('',(-0.943451111610983,0.,-1.82));
#15998=CARTESIAN_POINT('Origin',(0.,1.65,0.));
#15999=CARTESIAN_POINT('Origin',(0.,-1.85,0.));
#16000=CARTESIAN_POINT('',(0.,-1.85,-1.82));
#16001=CARTESIAN_POINT('Origin',(0.,-1.65,0.));
#16002=CARTESIAN_POINT('',(2.12781578149989,-1.65,-1.82));
#16003=CARTESIAN_POINT('',(0.,-1.65,-1.82));
#16004=CARTESIAN_POINT('',(-2.12781578149989,-1.65,-1.82));
#16005=CARTESIAN_POINT('Origin',(0.,-1.65,0.));
#16006=CARTESIAN_POINT('',(0.,-1.65,-1.82));
#16007=CARTESIAN_POINT('Origin',(0.,0.,0.));
#16008=CARTESIAN_POINT('',(-1.43895998899814E-16,-1.76221774462768E-32,
-2.35));
#16009=CARTESIAN_POINT('',(-1.43895998899814E-16,-1.76221774462768E-32,
2.35));
#16010=CARTESIAN_POINT('Origin',(0.,0.,0.));
#16011=CARTESIAN_POINT('Origin',(0.,1.55,-1.335));
#16012=CARTESIAN_POINT('',(-3.75878787878788,1.55,-1.82));
#16013=CARTESIAN_POINT('',(-2.12781578149989,1.55,-1.82));
#16014=CARTESIAN_POINT('',(0.,1.55,-1.82));
#16015=CARTESIAN_POINT('',(-2.51385336103051,1.55,-1.23310229877152));
#16016=CARTESIAN_POINT('',(-1.68,1.55,-0.84));
#16017=CARTESIAN_POINT('Origin',(0.,1.55,0.));
#16018=CARTESIAN_POINT('Origin',(0.,1.55,-1.335));
#16019=CARTESIAN_POINT('',(2.12781578149989,1.55,-1.82));
#16020=CARTESIAN_POINT('',(3.75878787878788,1.55,-1.82));
#16021=CARTESIAN_POINT('',(0.,1.55,-1.82));
#16022=CARTESIAN_POINT('',(2.51385336103051,1.55,-1.23310229877152));
#16023=CARTESIAN_POINT('Origin',(0.,1.55,0.));
#16024=CARTESIAN_POINT('',(3.78,1.55,-1.83));
#16025=CARTESIAN_POINT('Origin',(0.,-1.55,-1.335));
#16026=CARTESIAN_POINT('',(-2.12781578149989,-1.55,-1.82));
#16027=CARTESIAN_POINT('',(-3.75878787878788,-1.55,-1.82));
#16028=CARTESIAN_POINT('',(0.,-1.55,-1.82));
#16029=CARTESIAN_POINT('',(-2.51385336103051,-1.55,-1.23310229877152));
#16030=CARTESIAN_POINT('Origin',(0.,-1.55,0.));
#16031=CARTESIAN_POINT('',(-1.68,-1.55,-0.84));
#16032=CARTESIAN_POINT('Origin',(-3.78,0.,-1.83));
#16033=CARTESIAN_POINT('',(-3.75878787878788,0.,-1.82));
#16034=CARTESIAN_POINT('',(-2.51385336103051,0.,-1.23310229877152));
#16035=CARTESIAN_POINT('Origin',(0.,-1.55,-1.335));
#16036=CARTESIAN_POINT('',(3.75878787878788,-1.55,-1.82));
#16037=CARTESIAN_POINT('',(2.12781578149989,-1.55,-1.82));
#16038=CARTESIAN_POINT('',(0.,-1.55,-1.82));
#16039=CARTESIAN_POINT('',(2.51385336103051,-1.55,-1.23310229877152));
#16040=CARTESIAN_POINT('',(3.78,-1.55,-1.83));
#16041=CARTESIAN_POINT('Origin',(0.,-1.55,0.));
#16042=CARTESIAN_POINT('Origin',(1.68,0.,-0.84));
#16043=CARTESIAN_POINT('',(3.75878787878788,0.,-1.82));
#16044=CARTESIAN_POINT('',(2.51385336103051,0.,-1.23310229877153));
#16045=CARTESIAN_POINT('Origin',(0.,0.,-1.82));
#16046=CARTESIAN_POINT('',(-6.35,1.9,-1.82));
#16047=CARTESIAN_POINT('',(-6.35,-1.9,-1.82));
#16048=CARTESIAN_POINT('',(-6.35,1.9,-1.82));
#16049=CARTESIAN_POINT('',(6.35,-1.9,-1.82));
#16050=CARTESIAN_POINT('',(-6.35,-1.9,-1.82));
#16051=CARTESIAN_POINT('',(6.35,1.9,-1.82));
#16052=CARTESIAN_POINT('',(6.35,-1.9,-1.82));
#16053=CARTESIAN_POINT('',(6.35,1.9,-1.82));
#16054=CARTESIAN_POINT('',(-2.12781578149989,0.,-1.82));
#16055=CARTESIAN_POINT('',(-2.12781578149989,1.65,-1.82));
#16056=CARTESIAN_POINT('',(-2.12781578149989,0.,-1.82));
#16057=CARTESIAN_POINT('',(0.,1.65,-1.82));
#16058=CARTESIAN_POINT('',(2.12781578149989,1.65,-1.82));
#16059=CARTESIAN_POINT('',(0.,1.65,-1.82));
#16060=CARTESIAN_POINT('',(2.12781578149989,0.,-1.82));
#16061=CARTESIAN_POINT('',(2.12781578149989,0.,-1.82));
#16062=CARTESIAN_POINT('',(4.1,7.9602041944578E-17,-1.82));
#16063=CARTESIAN_POINT('Origin',(4.75,0.,-1.82));
#16064=CARTESIAN_POINT('',(-5.4,7.9602041944578E-17,-1.82));
#16065=CARTESIAN_POINT('Origin',(-4.75,0.,-1.82));
#16066=CARTESIAN_POINT('Origin',(0.,0.,0.));
#16067=CARTESIAN_POINT('',(-1.22049170419139,-1.4,-2.52));
#16068=CARTESIAN_POINT('',(1.22049170419139,-1.4,-2.52));
#16069=CARTESIAN_POINT('Origin',(0.,-1.4,0.));
#16070=CARTESIAN_POINT('',(-1.22049170419139,1.4,-2.52));
#16071=CARTESIAN_POINT('',(-1.22049170419139,0.,-2.52));
#16072=CARTESIAN_POINT('',(1.22049170419139,1.4,-2.52));
#16073=CARTESIAN_POINT('Origin',(0.,1.4,0.));
#16074=CARTESIAN_POINT('',(1.22049170419139,0.,-2.52));
#16075=CARTESIAN_POINT('Origin',(0.,0.,0.));
#16076=CARTESIAN_POINT('Origin',(0.,1.65,0.));
#16077=CARTESIAN_POINT('Origin',(0.,1.65,0.));
#16078=CARTESIAN_POINT('Origin',(3.35,1.4,-3.02));
#16079=CARTESIAN_POINT('',(-3.35,1.4,-2.52));
#16080=CARTESIAN_POINT('',(3.35,1.4,-2.52));
#16081=CARTESIAN_POINT('',(-3.35,1.4,-3.02));
#16082=CARTESIAN_POINT('',(-3.35,1.4,-3.02));
#16083=CARTESIAN_POINT('',(3.35,1.4,-3.02));
#16084=CARTESIAN_POINT('',(1.675,1.4,-3.02));
#16085=CARTESIAN_POINT('',(3.35,1.4,-2.52));
#16086=CARTESIAN_POINT('',(3.35,1.4,-3.02));
#16087=CARTESIAN_POINT('',(3.35,1.4,-2.52));
#16088=CARTESIAN_POINT('Origin',(0.,0.,-2.52));
#16089=CARTESIAN_POINT('',(-3.35,-1.4,-2.52));
#16090=CARTESIAN_POINT('',(-3.35,-1.4,-2.52));
#16091=CARTESIAN_POINT('',(-3.35,1.4,-2.52));
#16092=CARTESIAN_POINT('Origin',(3.35,-1.4,-3.02));
#16093=CARTESIAN_POINT('',(3.35,-1.4,-3.02));
#16094=CARTESIAN_POINT('',(3.35,-0.7,-3.02));
#16095=CARTESIAN_POINT('',(3.35,-1.4,-2.52));
#16096=CARTESIAN_POINT('',(3.35,-1.4,-3.02));
#16097=CARTESIAN_POINT('',(3.35,-1.4,-2.52));
#16098=CARTESIAN_POINT('Origin',(-3.35,-1.4,-3.02));
#16099=CARTESIAN_POINT('',(-3.35,-1.4,-2.52));
#16100=CARTESIAN_POINT('',(-3.35,-1.4,-3.02));
#16101=CARTESIAN_POINT('',(-1.675,-1.4,-3.02));
#16102=CARTESIAN_POINT('',(-3.35,-1.4,-3.02));
#16103=CARTESIAN_POINT('Origin',(-3.35,1.4,-3.02));
#16104=CARTESIAN_POINT('',(-3.35,0.7,-3.02));
#16105=CARTESIAN_POINT('Origin',(0.,0.,-2.52));
#16106=CARTESIAN_POINT('Origin',(-4.75,0.,-3.02));
#16107=CARTESIAN_POINT('',(-5.4,-7.9602041944578E-17,-3.02));
#16108=CARTESIAN_POINT('Origin',(-4.75,0.,-3.02));
#16109=CARTESIAN_POINT('',(-5.4,-7.9602041944578E-17,-3.02));
#16110=CARTESIAN_POINT('Origin',(4.75,0.,-3.02));
#16111=CARTESIAN_POINT('',(4.1,-7.9602041944578E-17,-3.02));
#16112=CARTESIAN_POINT('Origin',(4.75,0.,-3.02));
#16113=CARTESIAN_POINT('',(4.1,-7.9602041944578E-17,-3.02));
#16114=CARTESIAN_POINT('Origin',(6.35,1.9,-3.02));
#16115=CARTESIAN_POINT('',(6.35,1.9,-3.02));
#16116=CARTESIAN_POINT('',(-6.35,1.9,-3.02));
#16117=CARTESIAN_POINT('',(6.35,1.9,-3.02));
#16118=CARTESIAN_POINT('',(-6.35,1.9,-3.02));
#16119=CARTESIAN_POINT('',(6.35,1.9,-3.02));
#16120=CARTESIAN_POINT('Origin',(6.35,-1.9,-3.02));
#16121=CARTESIAN_POINT('',(6.35,-1.9,-3.02));
#16122=CARTESIAN_POINT('',(6.35,-1.9,-3.02));
#16123=CARTESIAN_POINT('',(6.35,-1.9,-3.02));
#16124=CARTESIAN_POINT('Origin',(-6.35,-1.9,-3.02));
#16125=CARTESIAN_POINT('',(-6.35,-1.9,-3.02));
#16126=CARTESIAN_POINT('',(-6.35,-1.9,-3.02));
#16127=CARTESIAN_POINT('',(-6.35,-1.9,-3.02));
#16128=CARTESIAN_POINT('Origin',(-6.35,1.9,-3.02));
#16129=CARTESIAN_POINT('',(-6.35,1.9,-3.02));
#16130=CARTESIAN_POINT('Origin',(0.,0.,-3.02));
#19302=UNCERTAINTY_MEASURE_WITH_UNIT(LENGTH_MEASURE(0.001),#19362,
'DISTANCE_ACCURACY_VALUE',
'Maximum model space distance between geometric entities at asserted c
onnectivities');
#19323=UNCERTAINTY_MEASURE_WITH_UNIT(LENGTH_MEASURE(0.001),#19362,
'DISTANCE_ACCURACY_VALUE',
'Maximum model space distance between geometric entities at asserted c
onnectivities');
#19340=(
GEOMETRIC_REPRESENTATION_CONTEXT(3)
GLOBAL_UNCERTAINTY_ASSIGNED_CONTEXT((#19302))
GLOBAL_UNIT_ASSIGNED_CONTEXT((#19362,#19364,#19365))
REPRESENTATION_CONTEXT('','3D')
);
#19361=(
GEOMETRIC_REPRESENTATION_CONTEXT(3)
GLOBAL_UNCERTAINTY_ASSIGNED_CONTEXT((#19323))
GLOBAL_UNIT_ASSIGNED_CONTEXT((#19362,#19364,#19365))
REPRESENTATION_CONTEXT('','3D')
);
#19362=(
LENGTH_UNIT()
NAMED_UNIT(*)
SI_UNIT(.CENTI.,.METRE.)
);
#19364=(
NAMED_UNIT(*)
PLANE_ANGLE_UNIT()
SI_UNIT($,.RADIAN.)
);
#19365=(
NAMED_UNIT(*)
SI_UNIT($,.STERADIAN.)
SOLID_ANGLE_UNIT()
);
#19382=SHAPE_DEFINITION_REPRESENTATION(#19419,#19504);
#19419=PRODUCT_DEFINITION_SHAPE('',$,#19542);
#19504=SHAPE_REPRESENTATION('',(#11579),#19340);
#19525=PRODUCT_DEFINITION_CONTEXT('part definition',#19638,'design');
#19542=PRODUCT_DEFINITION('Housing','Housing',#19579,#19525);
#19579=PRODUCT_DEFINITION_FORMATION('',$,#19656);
#19638=APPLICATION_CONTEXT(
'Core Data for Automotive Mechanical Design Process');
#19639=PRODUCT_CONTEXT('part definition',#19638,'mechanical');
#19656=PRODUCT('Housing','Housing','Housing',(#19639));
#19719=COLOUR_RGB('Dark Blue',0.08,0.2,0.34);
#19720=FILL_AREA_STYLE_COLOUR('',#19719);
#19721=FILL_AREA_STYLE('',(#19720));
#19722=SURFACE_STYLE_FILL_AREA(#19721);
#19723=SURFACE_SIDE_STYLE('',(#19722));
#19724=SURFACE_STYLE_USAGE(.BOTH.,#19723);
#19725=PRESENTATION_STYLE_ASSIGNMENT((#19724));
ENDSEC;
END-ISO-10303-21;
